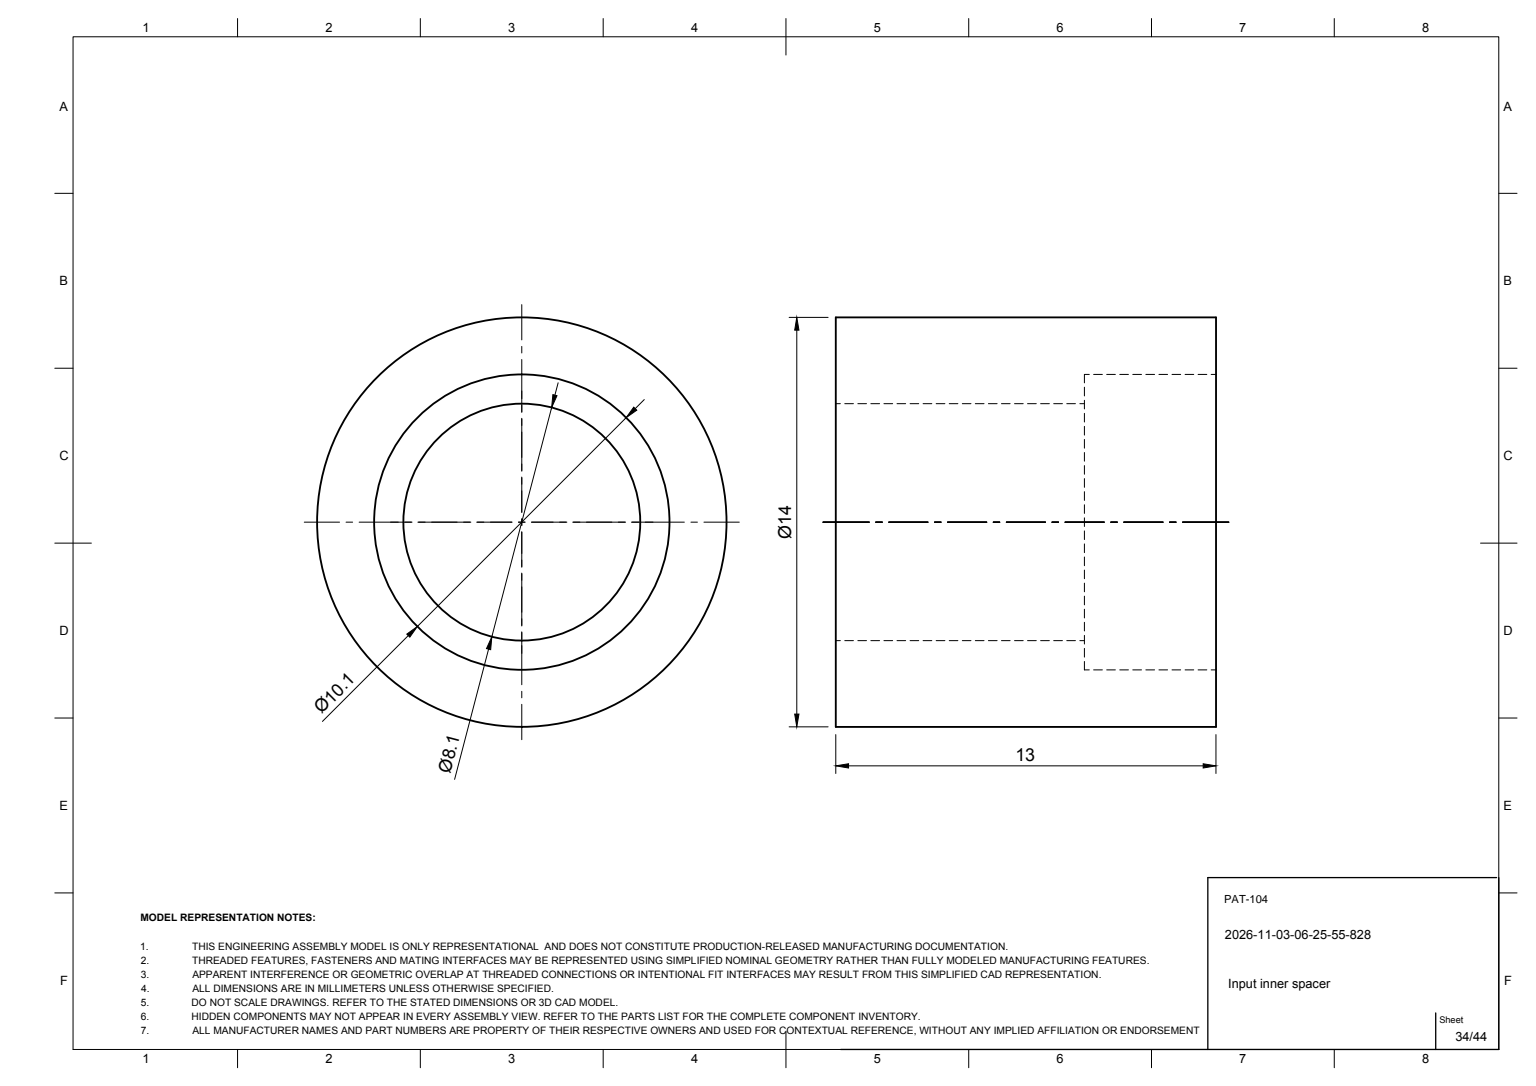
ISO-10303-21;
HEADER;
/* Generated by software containing ST-Developer
 * from STEP Tools, Inc. (www.steptools.com) 
 */

FILE_DESCRIPTION(
/* description */ ('Timing belt drive module 2 mm Pitch Timing 20T-40T'),

/* implementation_level */ '2;1');

FILE_NAME(
/* name */ 'Input inner spacer.step',
/* time_stamp */ '2026-10-28T03:25:12-07:00',
/* author */ (''),
/* organization */ (''),
/* preprocessor_version */ 'ST-DEVELOPER v20.2',
/* originating_system */ 'Autodesk Translation Framework v15.17.0.0',
/* authorisation */ '');

FILE_SCHEMA (('AUTOMOTIVE_DESIGN { 1 0 10303 214 3 1 1 }'));
ENDSEC;

DATA;
#10=MECHANICAL_DESIGN_GEOMETRIC_PRESENTATION_REPRESENTATION('',(#568),#17830);
#467=SHAPE_REPRESENTATION_RELATIONSHIP('SRR','None',#18040,#510);
#510=ADVANCED_BREP_SHAPE_REPRESENTATION('',(#624),#17815);
#568=STYLED_ITEM('',(#18331),#624);
#624=MANIFOLD_SOLID_BREP('Body1',#9027);
#734=FACE_BOUND('',#1893,.T.);
#735=FACE_BOUND('',#1897,.T.);
#736=FACE_BOUND('',#1899,.T.);
#915=PLANE('',#10219);
#916=PLANE('',#10226);
#917=PLANE('',#10227);
#1273=FACE_OUTER_BOUND('',#1891,.T.);
#1274=FACE_OUTER_BOUND('',#1892,.T.);
#1275=FACE_OUTER_BOUND('',#1894,.T.);
#1276=FACE_OUTER_BOUND('',#1895,.T.);
#1277=FACE_OUTER_BOUND('',#1896,.T.);
#1278=FACE_OUTER_BOUND('',#1898,.T.);
#1891=EDGE_LOOP('',(#7111,#7112,#7113,#7114));
#1892=EDGE_LOOP('',(#7115));
#1893=EDGE_LOOP('',(#7116));
#1894=EDGE_LOOP('',(#7117,#7118,#7119,#7120));
#1895=EDGE_LOOP('',(#7121,#7122,#7123,#7124));
#1896=EDGE_LOOP('',(#7125));
#1897=EDGE_LOOP('',(#7126));
#1898=EDGE_LOOP('',(#7127));
#1899=EDGE_LOOP('',(#7128));
#2484=CIRCLE('',#10217,0.505);
#2485=CIRCLE('',#10218,0.505);
#2486=CIRCLE('',#10220,0.405);
#2487=CIRCLE('',#10222,0.405);
#2488=CIRCLE('',#10224,0.7);
#2489=CIRCLE('',#10225,0.7);
#3083=LINE('',#15995,#3561);
#3084=LINE('',#16002,#3562);
#3085=LINE('',#16008,#3563);
#3561=VECTOR('',#12506,0.505);
#3562=VECTOR('',#12515,0.405);
#3563=VECTOR('',#12522,0.7);
#4207=VERTEX_POINT('',#15992);
#4208=VERTEX_POINT('',#15994);
#4209=VERTEX_POINT('',#15998);
#4210=VERTEX_POINT('',#16001);
#4211=VERTEX_POINT('',#16005);
#4212=VERTEX_POINT('',#16007);
#5238=EDGE_CURVE('',#4207,#4207,#2484,.T.);
#5239=EDGE_CURVE('',#4207,#4208,#3083,.T.);
#5240=EDGE_CURVE('',#4208,#4208,#2485,.T.);
#5241=EDGE_CURVE('',#4209,#4209,#2486,.T.);
#5242=EDGE_CURVE('',#4209,#4210,#3084,.T.);
#5243=EDGE_CURVE('',#4210,#4210,#2487,.T.);
#5244=EDGE_CURVE('',#4211,#4211,#2488,.T.);
#5245=EDGE_CURVE('',#4211,#4212,#3085,.T.);
#5246=EDGE_CURVE('',#4212,#4212,#2489,.T.);
#7111=ORIENTED_EDGE('',*,*,#5238,.F.);
#7112=ORIENTED_EDGE('',*,*,#5239,.T.);
#7113=ORIENTED_EDGE('',*,*,#5240,.F.);
#7114=ORIENTED_EDGE('',*,*,#5239,.F.);
#7115=ORIENTED_EDGE('',*,*,#5238,.T.);
#7116=ORIENTED_EDGE('',*,*,#5241,.F.);
#7117=ORIENTED_EDGE('',*,*,#5241,.T.);
#7118=ORIENTED_EDGE('',*,*,#5242,.T.);
#7119=ORIENTED_EDGE('',*,*,#5243,.T.);
#7120=ORIENTED_EDGE('',*,*,#5242,.F.);
#7121=ORIENTED_EDGE('',*,*,#5244,.F.);
#7122=ORIENTED_EDGE('',*,*,#5245,.T.);
#7123=ORIENTED_EDGE('',*,*,#5246,.T.);
#7124=ORIENTED_EDGE('',*,*,#5245,.F.);
#7125=ORIENTED_EDGE('',*,*,#5244,.T.);
#7126=ORIENTED_EDGE('',*,*,#5240,.T.);
#7127=ORIENTED_EDGE('',*,*,#5246,.F.);
#7128=ORIENTED_EDGE('',*,*,#5243,.F.);
#8301=CYLINDRICAL_SURFACE('',#10216,0.505);
#8302=CYLINDRICAL_SURFACE('',#10221,0.405);
#8303=CYLINDRICAL_SURFACE('',#10223,0.7);
#8771=ADVANCED_FACE('',(#1273),#8301,.F.);
#8772=ADVANCED_FACE('',(#1274,#734),#915,.T.);
#8773=ADVANCED_FACE('',(#1275),#8302,.F.);
#8774=ADVANCED_FACE('',(#1276),#8303,.T.);
#8775=ADVANCED_FACE('',(#1277,#735),#916,.T.);
#8776=ADVANCED_FACE('',(#1278,#736),#917,.F.);
#9027=CLOSED_SHELL('',(#8771,#8772,#8773,#8774,#8775,#8776));
#10215=AXIS2_PLACEMENT_3D('',#15990,#12500,#12501);
#10216=AXIS2_PLACEMENT_3D('',#15991,#12502,#12503);
#10217=AXIS2_PLACEMENT_3D('',#15993,#12504,#12505);
#10218=AXIS2_PLACEMENT_3D('',#15996,#12507,#12508);
#10219=AXIS2_PLACEMENT_3D('',#15997,#12509,#12510);
#10220=AXIS2_PLACEMENT_3D('',#15999,#12511,#12512);
#10221=AXIS2_PLACEMENT_3D('',#16000,#12513,#12514);
#10222=AXIS2_PLACEMENT_3D('',#16003,#12516,#12517);
#10223=AXIS2_PLACEMENT_3D('',#16004,#12518,#12519);
#10224=AXIS2_PLACEMENT_3D('',#16006,#12520,#12521);
#10225=AXIS2_PLACEMENT_3D('',#16009,#12523,#12524);
#10226=AXIS2_PLACEMENT_3D('',#16010,#12525,#12526);
#10227=AXIS2_PLACEMENT_3D('',#16011,#12527,#12528);
#12500=DIRECTION('axis',(0.,0.,1.));
#12501=DIRECTION('refdir',(1.,0.,0.));
#12502=DIRECTION('center_axis',(0.,1.,0.));
#12503=DIRECTION('ref_axis',(1.,0.,0.));
#12504=DIRECTION('center_axis',(0.,1.,0.));
#12505=DIRECTION('ref_axis',(1.,0.,0.));
#12506=DIRECTION('',(0.,1.,0.));
#12507=DIRECTION('center_axis',(0.,-1.,0.));
#12508=DIRECTION('ref_axis',(1.,0.,0.));
#12509=DIRECTION('center_axis',(0.,1.,0.));
#12510=DIRECTION('ref_axis',(1.,0.,0.));
#12511=DIRECTION('center_axis',(0.,1.,0.));
#12512=DIRECTION('ref_axis',(1.,0.,0.));
#12513=DIRECTION('center_axis',(0.,1.,0.));
#12514=DIRECTION('ref_axis',(1.,0.,0.));
#12515=DIRECTION('',(0.,-1.,0.));
#12516=DIRECTION('center_axis',(0.,-1.,0.));
#12517=DIRECTION('ref_axis',(1.,0.,0.));
#12518=DIRECTION('center_axis',(0.,1.,0.));
#12519=DIRECTION('ref_axis',(1.,0.,0.));
#12520=DIRECTION('center_axis',(0.,1.,0.));
#12521=DIRECTION('ref_axis',(1.,0.,0.));
#12522=DIRECTION('',(0.,-1.,0.));
#12523=DIRECTION('center_axis',(0.,1.,0.));
#12524=DIRECTION('ref_axis',(1.,0.,0.));
#12525=DIRECTION('center_axis',(0.,1.,0.));
#12526=DIRECTION('ref_axis',(1.,0.,0.));
#12527=DIRECTION('center_axis',(0.,1.,0.));
#12528=DIRECTION('ref_axis',(1.,0.,0.));
#15990=CARTESIAN_POINT('',(0.,0.,0.));
#15991=CARTESIAN_POINT('Origin',(0.,-1.8,7.));
#15992=CARTESIAN_POINT('',(-0.505,-1.8,7.));
#15993=CARTESIAN_POINT('Origin',(0.,-1.8,7.));
#15994=CARTESIAN_POINT('',(-0.505,-1.35,7.));
#15995=CARTESIAN_POINT('',(-0.505,-1.8,7.));
#15996=CARTESIAN_POINT('Origin',(0.,-1.35,7.));
#15997=CARTESIAN_POINT('Origin',(0.,-1.8,7.));
#15998=CARTESIAN_POINT('',(-0.405,-1.8,7.));
#15999=CARTESIAN_POINT('Origin',(0.,-1.8,7.));
#16000=CARTESIAN_POINT('Origin',(0.,-2.65,7.));
#16001=CARTESIAN_POINT('',(-0.405,-2.65,7.));
#16002=CARTESIAN_POINT('',(-0.405,-2.65,7.));
#16003=CARTESIAN_POINT('Origin',(0.,-2.65,7.));
#16004=CARTESIAN_POINT('Origin',(0.,-2.65,7.));
#16005=CARTESIAN_POINT('',(-0.7,-1.35,7.));
#16006=CARTESIAN_POINT('Origin',(0.,-1.35,7.));
#16007=CARTESIAN_POINT('',(-0.7,-2.65,7.));
#16008=CARTESIAN_POINT('',(-0.7,-2.65,7.));
#16009=CARTESIAN_POINT('Origin',(0.,-2.65,7.));
#16010=CARTESIAN_POINT('Origin',(0.,-1.35,7.));
#16011=CARTESIAN_POINT('Origin',(0.,-2.65,7.));
#17765=UNCERTAINTY_MEASURE_WITH_UNIT(LENGTH_MEASURE(0.001),#17831,
'DISTANCE_ACCURACY_VALUE',
'Maximum model space distance between geometric entities at asserted c
onnectivities');
#17780=UNCERTAINTY_MEASURE_WITH_UNIT(LENGTH_MEASURE(0.001),#17831,
'DISTANCE_ACCURACY_VALUE',
'Maximum model space distance between geometric entities at asserted c
onnectivities');
#17815=(
GEOMETRIC_REPRESENTATION_CONTEXT(3)
GLOBAL_UNCERTAINTY_ASSIGNED_CONTEXT((#17765))
GLOBAL_UNIT_ASSIGNED_CONTEXT((#17831,#17833,#17834))
REPRESENTATION_CONTEXT('','3D')
);
#17830=(
GEOMETRIC_REPRESENTATION_CONTEXT(3)
GLOBAL_UNCERTAINTY_ASSIGNED_CONTEXT((#17780))
GLOBAL_UNIT_ASSIGNED_CONTEXT((#17831,#17833,#17834))
REPRESENTATION_CONTEXT('','3D')
);
#17831=(
LENGTH_UNIT()
NAMED_UNIT(*)
SI_UNIT(.CENTI.,.METRE.)
);
#17833=(
NAMED_UNIT(*)
PLANE_ANGLE_UNIT()
SI_UNIT($,.RADIAN.)
);
#17834=(
NAMED_UNIT(*)
SI_UNIT($,.STERADIAN.)
SOLID_ANGLE_UNIT()
);
#17869=SHAPE_DEFINITION_REPRESENTATION(#17928,#18040);
#17928=PRODUCT_DEFINITION_SHAPE('',$,#18090);
#18040=SHAPE_REPRESENTATION('',(#10215),#17815);
#18055=PRODUCT_DEFINITION_CONTEXT('part definition',#18204,'design');
#18090=PRODUCT_DEFINITION('Input inner spacer','Input inner spacer',#18139,
#18055);
#18139=PRODUCT_DEFINITION_FORMATION('',$,#18240);
#18204=APPLICATION_CONTEXT(
'Core Data for Automotive Mechanical Design Process');
#18205=PRODUCT_CONTEXT('part definition',#18204,'mechanical');
#18240=PRODUCT('Input inner spacer','Input inner spacer',
'Input inner spacer',(#18205));
#18325=COLOUR_RGB('Off White',0.89,0.88,0.83);
#18326=FILL_AREA_STYLE_COLOUR('',#18325);
#18327=FILL_AREA_STYLE('',(#18326));
#18328=SURFACE_STYLE_FILL_AREA(#18327);
#18329=SURFACE_SIDE_STYLE('',(#18328));
#18330=SURFACE_STYLE_USAGE(.BOTH.,#18329);
#18331=PRESENTATION_STYLE_ASSIGNMENT((#18330));
ENDSEC;
END-ISO-10303-21;
